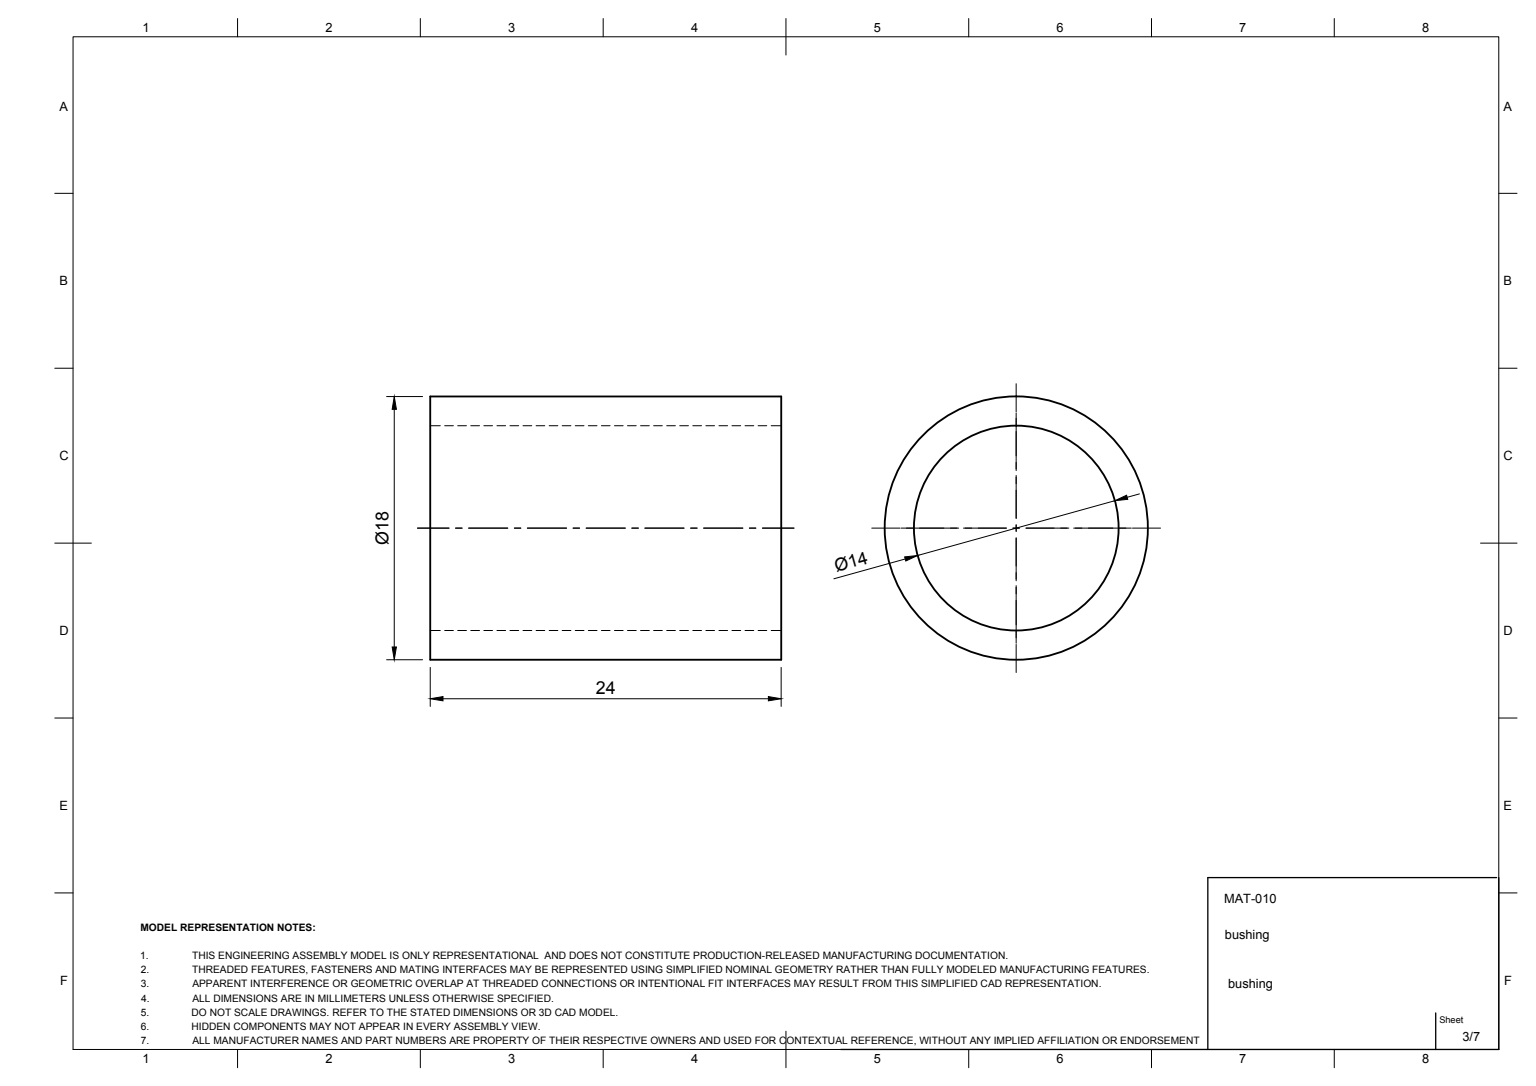
ISO-10303-21;
HEADER;
/* Generated by software containing ST-Developer
 * from STEP Tools, Inc. (www.steptools.com) 
 */

FILE_DESCRIPTION(
/* description */ ('STEP AP214'),
/* implementation_level */ '2;1');

FILE_NAME(
/* name */ 'Bushing.step',
/* time_stamp */ '2026-11-14T05:50:49-08:00',
/* author */ (''),
/* organization */ (''),
/* preprocessor_version */ 'ST-DEVELOPER v20.2',
/* originating_system */ 'Autodesk Translation Framework v15.17.0.0',
/* authorisation */ '');

FILE_SCHEMA (('AUTOMOTIVE_DESIGN { 1 0 10303 214 3 1 1 }'));
ENDSEC;

DATA;
#10=MECHANICAL_DESIGN_GEOMETRIC_PRESENTATION_REPRESENTATION('',(#157),#9903);
#143=SHAPE_REPRESENTATION_RELATIONSHIP('SRR','None',#9938,#150);
#150=ADVANCED_BREP_SHAPE_REPRESENTATION('',(#164),#9896);
#157=STYLED_ITEM('',(#9982),#164);
#164=MANIFOLD_SOLID_BREP('Body1',#2022);
#171=FACE_BOUND('',#373,.T.);
#172=FACE_BOUND('',#375,.T.);
#196=PLANE('',#2115);
#197=PLANE('',#2116);
#252=FACE_OUTER_BOUND('',#370,.T.);
#253=FACE_OUTER_BOUND('',#371,.T.);
#254=FACE_OUTER_BOUND('',#372,.T.);
#255=FACE_OUTER_BOUND('',#374,.T.);
#370=EDGE_LOOP('',(#1310,#1311,#1312,#1313));
#371=EDGE_LOOP('',(#1314,#1315,#1316,#1317));
#372=EDGE_LOOP('',(#1318));
#373=EDGE_LOOP('',(#1319));
#374=EDGE_LOOP('',(#1320));
#375=EDGE_LOOP('',(#1321));
#513=LINE('',#2882,#649);
#514=LINE('',#2888,#650);
#649=VECTOR('',#2326,7.);
#650=VECTOR('',#2333,9.);
#785=CIRCLE('',#2110,7.);
#786=CIRCLE('',#2111,7.);
#787=CIRCLE('',#2113,9.);
#788=CIRCLE('',#2114,9.);
#859=VERTEX_POINT('',#2879);
#860=VERTEX_POINT('',#2881);
#861=VERTEX_POINT('',#2885);
#862=VERTEX_POINT('',#2887);
#1036=EDGE_CURVE('',#859,#859,#785,.T.);
#1037=EDGE_CURVE('',#859,#860,#513,.T.);
#1038=EDGE_CURVE('',#860,#860,#786,.T.);
#1039=EDGE_CURVE('',#861,#861,#787,.T.);
#1040=EDGE_CURVE('',#861,#862,#514,.T.);
#1041=EDGE_CURVE('',#862,#862,#788,.T.);
#1310=ORIENTED_EDGE('',*,*,#1036,.T.);
#1311=ORIENTED_EDGE('',*,*,#1037,.T.);
#1312=ORIENTED_EDGE('',*,*,#1038,.F.);
#1313=ORIENTED_EDGE('',*,*,#1037,.F.);
#1314=ORIENTED_EDGE('',*,*,#1039,.T.);
#1315=ORIENTED_EDGE('',*,*,#1040,.T.);
#1316=ORIENTED_EDGE('',*,*,#1041,.F.);
#1317=ORIENTED_EDGE('',*,*,#1040,.F.);
#1318=ORIENTED_EDGE('',*,*,#1041,.T.);
#1319=ORIENTED_EDGE('',*,*,#1036,.F.);
#1320=ORIENTED_EDGE('',*,*,#1039,.F.);
#1321=ORIENTED_EDGE('',*,*,#1038,.T.);
#1858=CYLINDRICAL_SURFACE('',#2109,7.);
#1859=CYLINDRICAL_SURFACE('',#2112,9.);
#1904=ADVANCED_FACE('',(#252),#1858,.F.);
#1905=ADVANCED_FACE('',(#253),#1859,.T.);
#1906=ADVANCED_FACE('',(#254,#171),#196,.T.);
#1907=ADVANCED_FACE('',(#255,#172),#197,.F.);
#2022=CLOSED_SHELL('',(#1904,#1905,#1906,#1907));
#2108=AXIS2_PLACEMENT_3D('',#2877,#2320,#2321);
#2109=AXIS2_PLACEMENT_3D('',#2878,#2322,#2323);
#2110=AXIS2_PLACEMENT_3D('',#2880,#2324,#2325);
#2111=AXIS2_PLACEMENT_3D('',#2883,#2327,#2328);
#2112=AXIS2_PLACEMENT_3D('',#2884,#2329,#2330);
#2113=AXIS2_PLACEMENT_3D('',#2886,#2331,#2332);
#2114=AXIS2_PLACEMENT_3D('',#2889,#2334,#2335);
#2115=AXIS2_PLACEMENT_3D('',#2890,#2336,#2337);
#2116=AXIS2_PLACEMENT_3D('',#2891,#2338,#2339);
#2320=DIRECTION('axis',(0.,0.,1.));
#2321=DIRECTION('refdir',(1.,0.,0.));
#2322=DIRECTION('center_axis',(0.,0.,-1.));
#2323=DIRECTION('ref_axis',(-1.,0.,0.));
#2324=DIRECTION('center_axis',(0.,0.,1.));
#2325=DIRECTION('ref_axis',(1.,0.,0.));
#2326=DIRECTION('',(0.,0.,-1.));
#2327=DIRECTION('center_axis',(0.,0.,1.));
#2328=DIRECTION('ref_axis',(1.,0.,0.));
#2329=DIRECTION('center_axis',(0.,0.,-1.));
#2330=DIRECTION('ref_axis',(-1.,0.,0.));
#2331=DIRECTION('center_axis',(0.,0.,1.));
#2332=DIRECTION('ref_axis',(1.,0.,0.));
#2333=DIRECTION('',(0.,0.,1.));
#2334=DIRECTION('center_axis',(0.,0.,1.));
#2335=DIRECTION('ref_axis',(1.,0.,0.));
#2336=DIRECTION('center_axis',(0.,0.,1.));
#2337=DIRECTION('ref_axis',(1.,0.,0.));
#2338=DIRECTION('center_axis',(0.,0.,1.));
#2339=DIRECTION('ref_axis',(1.,0.,0.));
#2877=CARTESIAN_POINT('',(0.,0.,0.));
#2878=CARTESIAN_POINT('Origin',(0.,0.,24.));
#2879=CARTESIAN_POINT('',(7.,-8.57252759403147E-16,24.));
#2880=CARTESIAN_POINT('Origin',(0.,0.,24.));
#2881=CARTESIAN_POINT('',(7.,-8.57252759403147E-16,0.));
#2882=CARTESIAN_POINT('',(7.,-8.57252759403147E-16,24.));
#2883=CARTESIAN_POINT('Origin',(0.,0.,0.));
#2884=CARTESIAN_POINT('Origin',(0.,0.,24.));
#2885=CARTESIAN_POINT('',(9.,-1.10218211923262E-15,0.));
#2886=CARTESIAN_POINT('Origin',(0.,0.,0.));
#2887=CARTESIAN_POINT('',(9.,-1.10218211923262E-15,24.));
#2888=CARTESIAN_POINT('',(9.,-1.10218211923262E-15,24.));
#2889=CARTESIAN_POINT('Origin',(0.,0.,24.));
#2890=CARTESIAN_POINT('Origin',(0.,0.,24.));
#2891=CARTESIAN_POINT('Origin',(0.,0.,0.));
#9887=UNCERTAINTY_MEASURE_WITH_UNIT(LENGTH_MEASURE(0.01),#9904,
'DISTANCE_ACCURACY_VALUE',
'Maximum model space distance between geometric entities at asserted c
onnectivities');
#9894=UNCERTAINTY_MEASURE_WITH_UNIT(LENGTH_MEASURE(0.01),#9904,
'DISTANCE_ACCURACY_VALUE',
'Maximum model space distance between geometric entities at asserted c
onnectivities');
#9896=(
GEOMETRIC_REPRESENTATION_CONTEXT(3)
GLOBAL_UNCERTAINTY_ASSIGNED_CONTEXT((#9887))
GLOBAL_UNIT_ASSIGNED_CONTEXT((#9904,#9906,#9907))
REPRESENTATION_CONTEXT('','3D')
);
#9903=(
GEOMETRIC_REPRESENTATION_CONTEXT(3)
GLOBAL_UNCERTAINTY_ASSIGNED_CONTEXT((#9894))
GLOBAL_UNIT_ASSIGNED_CONTEXT((#9904,#9906,#9907))
REPRESENTATION_CONTEXT('','3D')
);
#9904=(
LENGTH_UNIT()
NAMED_UNIT(*)
SI_UNIT(.MILLI.,.METRE.)
);
#9906=(
NAMED_UNIT(*)
PLANE_ANGLE_UNIT()
SI_UNIT($,.RADIAN.)
);
#9907=(
NAMED_UNIT(*)
SI_UNIT($,.STERADIAN.)
SOLID_ANGLE_UNIT()
);
#9909=SHAPE_DEFINITION_REPRESENTATION(#9917,#9938);
#9917=PRODUCT_DEFINITION_SHAPE('',$,#9947);
#9938=SHAPE_REPRESENTATION('',(#2108),#9896);
#9945=PRODUCT_DEFINITION_CONTEXT('part definition',#9971,'design');
#9947=PRODUCT_DEFINITION('bushing','Bushing',#9955,#9945);
#9955=PRODUCT_DEFINITION_FORMATION('',$,#9974);
#9971=APPLICATION_CONTEXT(
'Core Data for Automotive Mechanical Design Process');
#9972=PRODUCT_CONTEXT('part definition',#9971,'mechanical');
#9974=PRODUCT('bushing','Bushing',$,(#9972));
#9982=PRESENTATION_STYLE_ASSIGNMENT((#9987));
#9987=SURFACE_STYLE_USAGE(.BOTH.,#9992);
#9992=SURFACE_SIDE_STYLE('',(#9997));
#9997=SURFACE_STYLE_FILL_AREA(#10002);
#10002=FILL_AREA_STYLE('Opaque(97,158,199)',(#10007));
#10007=FILL_AREA_STYLE_COLOUR('Opaque(97,158,199)',#10012);
#10012=COLOUR_RGB('Opaque(97,158,199)',0.380392156862745,0.619607843137255,
0.780392156862745);
ENDSEC;
END-ISO-10303-21;
